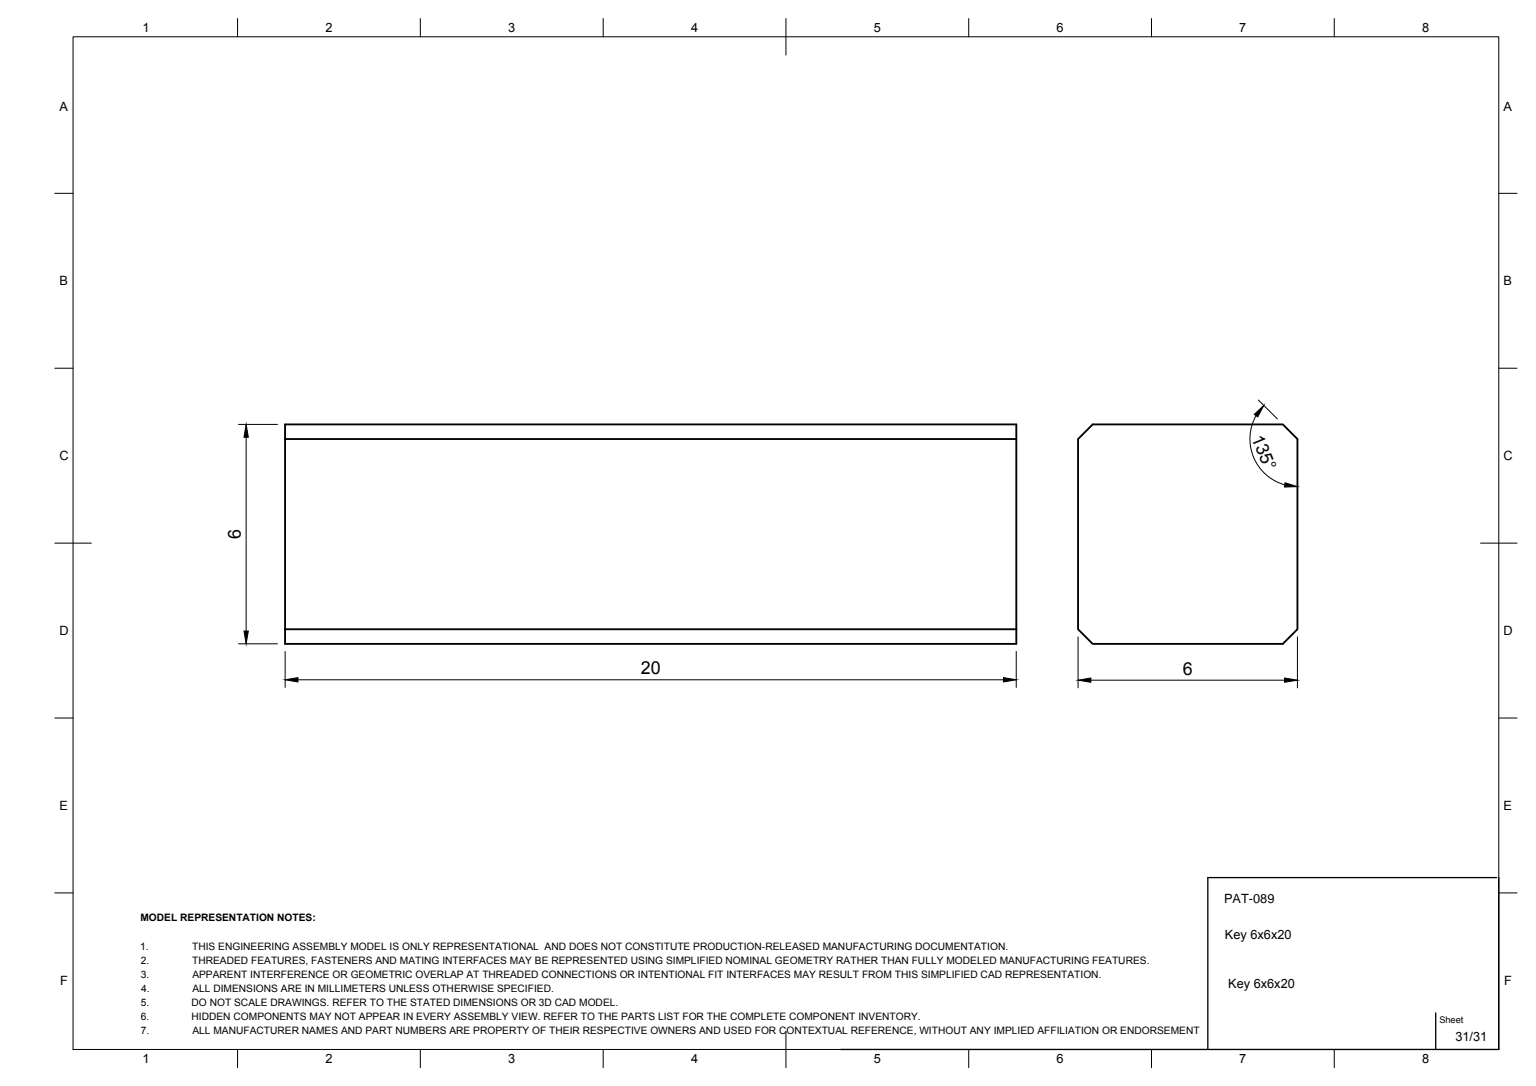
ISO-10303-21;
HEADER;
/* Generated by software containing ST-Developer
 * from STEP Tools, Inc. (www.steptools.com) 
 */

FILE_DESCRIPTION(
/* description */ ('Rotary union on bearing shaft'),
/* implementation_level */ '2;1');

FILE_NAME(
/* name */ 'Key 6x6x20.step',
/* time_stamp */ '2026-10-28T03:24:01-07:00',
/* author */ (''),
/* organization */ (''),
/* preprocessor_version */ 'ST-DEVELOPER v20.2',
/* originating_system */ 'Autodesk Translation Framework v15.17.0.0',
/* authorisation */ '');

FILE_SCHEMA (('AUTOMOTIVE_DESIGN { 1 0 10303 214 3 1 1 }'));
ENDSEC;

DATA;
#10=MECHANICAL_DESIGN_GEOMETRIC_PRESENTATION_REPRESENTATION('',(#346),#9448);
#284=SHAPE_REPRESENTATION_RELATIONSHIP('SRR','None',#9586,#311);
#311=ADVANCED_BREP_SHAPE_REPRESENTATION('',(#379),#9446);
#346=STYLED_ITEM('',(#9778),#379);
#379=MANIFOLD_SOLID_BREP('Body1',#4903);
#635=PLANE('',#5781);
#636=PLANE('',#5782);
#637=PLANE('',#5783);
#638=PLANE('',#5784);
#639=PLANE('',#5785);
#640=PLANE('',#5786);
#641=PLANE('',#5787);
#642=PLANE('',#5788);
#643=PLANE('',#5789);
#644=PLANE('',#5790);
#928=FACE_OUTER_BOUND('',#1333,.T.);
#929=FACE_OUTER_BOUND('',#1334,.T.);
#930=FACE_OUTER_BOUND('',#1335,.T.);
#931=FACE_OUTER_BOUND('',#1336,.T.);
#932=FACE_OUTER_BOUND('',#1337,.T.);
#933=FACE_OUTER_BOUND('',#1338,.T.);
#934=FACE_OUTER_BOUND('',#1339,.T.);
#935=FACE_OUTER_BOUND('',#1340,.T.);
#936=FACE_OUTER_BOUND('',#1341,.T.);
#937=FACE_OUTER_BOUND('',#1342,.T.);
#1333=EDGE_LOOP('',(#4367,#4368,#4369,#4370,#4371,#4372,#4373,#4374));
#1334=EDGE_LOOP('',(#4375,#4376,#4377,#4378));
#1335=EDGE_LOOP('',(#4379,#4380,#4381,#4382));
#1336=EDGE_LOOP('',(#4383,#4384,#4385,#4386));
#1337=EDGE_LOOP('',(#4387,#4388,#4389,#4390));
#1338=EDGE_LOOP('',(#4391,#4392,#4393,#4394,#4395,#4396,#4397,#4398));
#1339=EDGE_LOOP('',(#4399,#4400,#4401,#4402));
#1340=EDGE_LOOP('',(#4403,#4404,#4405,#4406));
#1341=EDGE_LOOP('',(#4407,#4408,#4409,#4410));
#1342=EDGE_LOOP('',(#4411,#4412,#4413,#4414));
#1633=LINE('',#9257,#1953);
#1634=LINE('',#9259,#1954);
#1635=LINE('',#9261,#1955);
#1636=LINE('',#9263,#1956);
#1637=LINE('',#9265,#1957);
#1638=LINE('',#9267,#1958);
#1639=LINE('',#9269,#1959);
#1640=LINE('',#9270,#1960);
#1641=LINE('',#9273,#1961);
#1642=LINE('',#9275,#1962);
#1643=LINE('',#9276,#1963);
#1644=LINE('',#9279,#1964);
#1645=LINE('',#9280,#1965);
#1646=LINE('',#9283,#1966);
#1647=LINE('',#9284,#1967);
#1648=LINE('',#9287,#1968);
#1649=LINE('',#9288,#1969);
#1650=LINE('',#9292,#1970);
#1651=LINE('',#9293,#1971);
#1652=LINE('',#9295,#1972);
#1653=LINE('',#9296,#1973);
#1654=LINE('',#9298,#1974);
#1655=LINE('',#9300,#1975);
#1656=LINE('',#9302,#1976);
#1953=VECTOR('',#7256,1.);
#1954=VECTOR('',#7257,1.);
#1955=VECTOR('',#7258,1.);
#1956=VECTOR('',#7259,1.);
#1957=VECTOR('',#7260,1.);
#1958=VECTOR('',#7261,1.);
#1959=VECTOR('',#7262,1.);
#1960=VECTOR('',#7263,1.);
#1961=VECTOR('',#7266,1.);
#1962=VECTOR('',#7267,1.);
#1963=VECTOR('',#7268,1.);
#1964=VECTOR('',#7271,1.);
#1965=VECTOR('',#7272,1.);
#1966=VECTOR('',#7275,1.);
#1967=VECTOR('',#7276,1.);
#1968=VECTOR('',#7279,1.);
#1969=VECTOR('',#7280,1.);
#1970=VECTOR('',#7283,1.);
#1971=VECTOR('',#7284,1.);
#1972=VECTOR('',#7285,1.);
#1973=VECTOR('',#7286,1.);
#1974=VECTOR('',#7289,1.);
#1975=VECTOR('',#7292,1.);
#1976=VECTOR('',#7295,1.);
#2625=VERTEX_POINT('',#9255);
#2626=VERTEX_POINT('',#9256);
#2627=VERTEX_POINT('',#9258);
#2628=VERTEX_POINT('',#9260);
#2629=VERTEX_POINT('',#9262);
#2630=VERTEX_POINT('',#9264);
#2631=VERTEX_POINT('',#9266);
#2632=VERTEX_POINT('',#9268);
#2633=VERTEX_POINT('',#9272);
#2634=VERTEX_POINT('',#9274);
#2635=VERTEX_POINT('',#9278);
#2636=VERTEX_POINT('',#9282);
#2637=VERTEX_POINT('',#9286);
#2638=VERTEX_POINT('',#9290);
#2639=VERTEX_POINT('',#9291);
#2640=VERTEX_POINT('',#9294);
#3211=EDGE_CURVE('',#2625,#2626,#1633,.T.);
#3212=EDGE_CURVE('',#2627,#2625,#1634,.T.);
#3213=EDGE_CURVE('',#2628,#2627,#1635,.T.);
#3214=EDGE_CURVE('',#2629,#2628,#1636,.T.);
#3215=EDGE_CURVE('',#2630,#2629,#1637,.T.);
#3216=EDGE_CURVE('',#2631,#2630,#1638,.T.);
#3217=EDGE_CURVE('',#2632,#2631,#1639,.T.);
#3218=EDGE_CURVE('',#2626,#2632,#1640,.T.);
#3219=EDGE_CURVE('',#2629,#2633,#1641,.T.);
#3220=EDGE_CURVE('',#2633,#2634,#1642,.T.);
#3221=EDGE_CURVE('',#2634,#2630,#1643,.T.);
#3222=EDGE_CURVE('',#2635,#2628,#1644,.T.);
#3223=EDGE_CURVE('',#2635,#2633,#1645,.T.);
#3224=EDGE_CURVE('',#2627,#2636,#1646,.T.);
#3225=EDGE_CURVE('',#2636,#2635,#1647,.T.);
#3226=EDGE_CURVE('',#2637,#2625,#1648,.T.);
#3227=EDGE_CURVE('',#2637,#2636,#1649,.T.);
#3228=EDGE_CURVE('',#2638,#2639,#1650,.T.);
#3229=EDGE_CURVE('',#2634,#2638,#1651,.T.);
#3230=EDGE_CURVE('',#2640,#2637,#1652,.T.);
#3231=EDGE_CURVE('',#2639,#2640,#1653,.T.);
#3232=EDGE_CURVE('',#2631,#2638,#1654,.T.);
#3233=EDGE_CURVE('',#2626,#2640,#1655,.T.);
#3234=EDGE_CURVE('',#2639,#2632,#1656,.T.);
#4367=ORIENTED_EDGE('',*,*,#3211,.F.);
#4368=ORIENTED_EDGE('',*,*,#3212,.F.);
#4369=ORIENTED_EDGE('',*,*,#3213,.F.);
#4370=ORIENTED_EDGE('',*,*,#3214,.F.);
#4371=ORIENTED_EDGE('',*,*,#3215,.F.);
#4372=ORIENTED_EDGE('',*,*,#3216,.F.);
#4373=ORIENTED_EDGE('',*,*,#3217,.F.);
#4374=ORIENTED_EDGE('',*,*,#3218,.F.);
#4375=ORIENTED_EDGE('',*,*,#3215,.T.);
#4376=ORIENTED_EDGE('',*,*,#3219,.T.);
#4377=ORIENTED_EDGE('',*,*,#3220,.T.);
#4378=ORIENTED_EDGE('',*,*,#3221,.T.);
#4379=ORIENTED_EDGE('',*,*,#3214,.T.);
#4380=ORIENTED_EDGE('',*,*,#3222,.F.);
#4381=ORIENTED_EDGE('',*,*,#3223,.T.);
#4382=ORIENTED_EDGE('',*,*,#3219,.F.);
#4383=ORIENTED_EDGE('',*,*,#3213,.T.);
#4384=ORIENTED_EDGE('',*,*,#3224,.T.);
#4385=ORIENTED_EDGE('',*,*,#3225,.T.);
#4386=ORIENTED_EDGE('',*,*,#3222,.T.);
#4387=ORIENTED_EDGE('',*,*,#3212,.T.);
#4388=ORIENTED_EDGE('',*,*,#3226,.F.);
#4389=ORIENTED_EDGE('',*,*,#3227,.T.);
#4390=ORIENTED_EDGE('',*,*,#3224,.F.);
#4391=ORIENTED_EDGE('',*,*,#3228,.F.);
#4392=ORIENTED_EDGE('',*,*,#3229,.F.);
#4393=ORIENTED_EDGE('',*,*,#3220,.F.);
#4394=ORIENTED_EDGE('',*,*,#3223,.F.);
#4395=ORIENTED_EDGE('',*,*,#3225,.F.);
#4396=ORIENTED_EDGE('',*,*,#3227,.F.);
#4397=ORIENTED_EDGE('',*,*,#3230,.F.);
#4398=ORIENTED_EDGE('',*,*,#3231,.F.);
#4399=ORIENTED_EDGE('',*,*,#3216,.T.);
#4400=ORIENTED_EDGE('',*,*,#3221,.F.);
#4401=ORIENTED_EDGE('',*,*,#3229,.T.);
#4402=ORIENTED_EDGE('',*,*,#3232,.F.);
#4403=ORIENTED_EDGE('',*,*,#3211,.T.);
#4404=ORIENTED_EDGE('',*,*,#3233,.T.);
#4405=ORIENTED_EDGE('',*,*,#3230,.T.);
#4406=ORIENTED_EDGE('',*,*,#3226,.T.);
#4407=ORIENTED_EDGE('',*,*,#3217,.T.);
#4408=ORIENTED_EDGE('',*,*,#3232,.T.);
#4409=ORIENTED_EDGE('',*,*,#3228,.T.);
#4410=ORIENTED_EDGE('',*,*,#3234,.T.);
#4411=ORIENTED_EDGE('',*,*,#3218,.T.);
#4412=ORIENTED_EDGE('',*,*,#3234,.F.);
#4413=ORIENTED_EDGE('',*,*,#3231,.T.);
#4414=ORIENTED_EDGE('',*,*,#3233,.F.);
#4841=ADVANCED_FACE('',(#928),#635,.F.);
#4842=ADVANCED_FACE('',(#929),#636,.T.);
#4843=ADVANCED_FACE('',(#930),#637,.T.);
#4844=ADVANCED_FACE('',(#931),#638,.T.);
#4845=ADVANCED_FACE('',(#932),#639,.T.);
#4846=ADVANCED_FACE('',(#933),#640,.T.);
#4847=ADVANCED_FACE('',(#934),#641,.F.);
#4848=ADVANCED_FACE('',(#935),#642,.T.);
#4849=ADVANCED_FACE('',(#936),#643,.T.);
#4850=ADVANCED_FACE('',(#937),#644,.T.);
#4903=CLOSED_SHELL('',(#4841,#4842,#4843,#4844,#4845,#4846,#4847,#4848,
#4849,#4850));
#5780=AXIS2_PLACEMENT_3D('',#9253,#7252,#7253);
#5781=AXIS2_PLACEMENT_3D('',#9254,#7254,#7255);
#5782=AXIS2_PLACEMENT_3D('',#9271,#7264,#7265);
#5783=AXIS2_PLACEMENT_3D('',#9277,#7269,#7270);
#5784=AXIS2_PLACEMENT_3D('',#9281,#7273,#7274);
#5785=AXIS2_PLACEMENT_3D('',#9285,#7277,#7278);
#5786=AXIS2_PLACEMENT_3D('',#9289,#7281,#7282);
#5787=AXIS2_PLACEMENT_3D('',#9297,#7287,#7288);
#5788=AXIS2_PLACEMENT_3D('',#9299,#7290,#7291);
#5789=AXIS2_PLACEMENT_3D('',#9301,#7293,#7294);
#5790=AXIS2_PLACEMENT_3D('',#9303,#7296,#7297);
#7252=DIRECTION('axis',(0.,0.,1.));
#7253=DIRECTION('refdir',(1.,0.,0.));
#7254=DIRECTION('center_axis',(1.,0.,0.));
#7255=DIRECTION('ref_axis',(0.,0.,-1.));
#7256=DIRECTION('',(0.,-0.707106781186547,-0.707106781186548));
#7257=DIRECTION('',(0.,-1.,0.));
#7258=DIRECTION('',(0.,-0.707106781186547,0.707106781186548));
#7259=DIRECTION('',(0.,0.,1.));
#7260=DIRECTION('',(0.,0.707106781186547,0.707106781186548));
#7261=DIRECTION('',(0.,1.,0.));
#7262=DIRECTION('',(0.,0.707106781186547,-0.707106781186548));
#7263=DIRECTION('',(0.,0.,-1.));
#7264=DIRECTION('center_axis',(0.,0.707106781186548,-0.707106781186547));
#7265=DIRECTION('ref_axis',(-1.,0.,0.));
#7266=DIRECTION('',(1.,0.,0.));
#7267=DIRECTION('',(0.,-0.707106781186547,-0.707106781186548));
#7268=DIRECTION('',(-1.,0.,0.));
#7269=DIRECTION('center_axis',(0.,1.,0.));
#7270=DIRECTION('ref_axis',(-1.,0.,0.));
#7271=DIRECTION('',(-1.,0.,0.));
#7272=DIRECTION('',(0.,0.,-1.));
#7273=DIRECTION('center_axis',(0.,0.707106781186548,0.707106781186547));
#7274=DIRECTION('ref_axis',(1.,0.,0.));
#7275=DIRECTION('',(1.,0.,0.));
#7276=DIRECTION('',(0.,0.707106781186547,-0.707106781186548));
#7277=DIRECTION('center_axis',(0.,0.,1.));
#7278=DIRECTION('ref_axis',(1.,0.,0.));
#7279=DIRECTION('',(-1.,0.,0.));
#7280=DIRECTION('',(0.,1.,0.));
#7281=DIRECTION('center_axis',(1.,0.,0.));
#7282=DIRECTION('ref_axis',(0.,0.,-1.));
#7283=DIRECTION('',(0.,-0.707106781186547,0.707106781186548));
#7284=DIRECTION('',(0.,-1.,0.));
#7285=DIRECTION('',(0.,0.707106781186547,0.707106781186548));
#7286=DIRECTION('',(0.,0.,1.));
#7287=DIRECTION('center_axis',(0.,0.,1.));
#7288=DIRECTION('ref_axis',(1.,0.,0.));
#7289=DIRECTION('',(1.,0.,0.));
#7290=DIRECTION('center_axis',(0.,-0.707106781186548,0.707106781186547));
#7291=DIRECTION('ref_axis',(1.,0.,0.));
#7292=DIRECTION('',(1.,0.,0.));
#7293=DIRECTION('center_axis',(0.,-0.707106781186548,-0.707106781186547));
#7294=DIRECTION('ref_axis',(-1.,0.,0.));
#7295=DIRECTION('',(-1.,0.,0.));
#7296=DIRECTION('center_axis',(0.,-1.,0.));
#7297=DIRECTION('ref_axis',(1.,0.,0.));
#9253=CARTESIAN_POINT('',(0.,0.,0.));
#9254=CARTESIAN_POINT('Origin',(-1.,0.,0.35));
#9255=CARTESIAN_POINT('',(-1.,-0.26,0.6));
#9256=CARTESIAN_POINT('',(-1.,-0.3,0.56));
#9257=CARTESIAN_POINT('',(-1.,-0.2675,0.5925));
#9258=CARTESIAN_POINT('',(-1.,0.26,0.6));
#9259=CARTESIAN_POINT('',(-1.,0.,0.6));
#9260=CARTESIAN_POINT('',(-1.,0.3,0.56));
#9261=CARTESIAN_POINT('',(-1.,0.2675,0.5925));
#9262=CARTESIAN_POINT('',(-1.,0.3,0.04));
#9263=CARTESIAN_POINT('',(-1.,0.3,0.175));
#9264=CARTESIAN_POINT('',(-1.,0.26,0.));
#9265=CARTESIAN_POINT('',(-1.,0.2925,0.0325));
#9266=CARTESIAN_POINT('',(-1.,-0.26,0.));
#9267=CARTESIAN_POINT('',(-1.,0.,0.));
#9268=CARTESIAN_POINT('',(-1.,-0.3,0.04));
#9269=CARTESIAN_POINT('',(-1.,-0.2925,0.0325));
#9270=CARTESIAN_POINT('',(-1.,-0.3,0.175));
#9271=CARTESIAN_POINT('Origin',(0.75,0.28,0.02));
#9272=CARTESIAN_POINT('',(1.,0.3,0.04));
#9273=CARTESIAN_POINT('',(0.75,0.3,0.04));
#9274=CARTESIAN_POINT('',(1.,0.26,0.));
#9275=CARTESIAN_POINT('',(1.,0.2925,0.0325));
#9276=CARTESIAN_POINT('',(0.75,0.26,0.));
#9277=CARTESIAN_POINT('Origin',(1.5,0.3,0.));
#9278=CARTESIAN_POINT('',(1.,0.3,0.56));
#9279=CARTESIAN_POINT('',(0.75,0.3,0.56));
#9280=CARTESIAN_POINT('',(1.,0.3,0.175));
#9281=CARTESIAN_POINT('Origin',(0.75,0.28,0.58));
#9282=CARTESIAN_POINT('',(1.,0.26,0.6));
#9283=CARTESIAN_POINT('',(0.75,0.26,0.6));
#9284=CARTESIAN_POINT('',(1.,0.2675,0.5925));
#9285=CARTESIAN_POINT('Origin',(0.,0.,0.6));
#9286=CARTESIAN_POINT('',(1.,-0.26,0.6));
#9287=CARTESIAN_POINT('',(-0.75,-0.26,0.6));
#9288=CARTESIAN_POINT('',(1.,0.,0.6));
#9289=CARTESIAN_POINT('Origin',(1.,0.,0.35));
#9290=CARTESIAN_POINT('',(1.,-0.26,0.));
#9291=CARTESIAN_POINT('',(1.,-0.3,0.04));
#9292=CARTESIAN_POINT('',(1.,-0.2925,0.0325));
#9293=CARTESIAN_POINT('',(1.,0.,0.));
#9294=CARTESIAN_POINT('',(1.,-0.3,0.56));
#9295=CARTESIAN_POINT('',(1.,-0.2675,0.5925));
#9296=CARTESIAN_POINT('',(1.,-0.3,0.175));
#9297=CARTESIAN_POINT('Origin',(0.,0.,0.));
#9298=CARTESIAN_POINT('',(-0.75,-0.26,0.));
#9299=CARTESIAN_POINT('Origin',(-0.75,-0.28,0.58));
#9300=CARTESIAN_POINT('',(-0.75,-0.3,0.56));
#9301=CARTESIAN_POINT('Origin',(-0.75,-0.28,0.02));
#9302=CARTESIAN_POINT('',(-0.75,-0.3,0.04));
#9303=CARTESIAN_POINT('Origin',(-1.5,-0.3,0.));
#9414=UNCERTAINTY_MEASURE_WITH_UNIT(LENGTH_MEASURE(0.001),#9449,
'DISTANCE_ACCURACY_VALUE',
'Maximum model space distance between geometric entities at asserted c
onnectivities');
#9416=UNCERTAINTY_MEASURE_WITH_UNIT(LENGTH_MEASURE(0.001),#9449,
'DISTANCE_ACCURACY_VALUE',
'Maximum model space distance between geometric entities at asserted c
onnectivities');
#9446=(
GEOMETRIC_REPRESENTATION_CONTEXT(3)
GLOBAL_UNCERTAINTY_ASSIGNED_CONTEXT((#9414))
GLOBAL_UNIT_ASSIGNED_CONTEXT((#9449,#9451,#9452))
REPRESENTATION_CONTEXT('','3D')
);
#9448=(
GEOMETRIC_REPRESENTATION_CONTEXT(3)
GLOBAL_UNCERTAINTY_ASSIGNED_CONTEXT((#9416))
GLOBAL_UNIT_ASSIGNED_CONTEXT((#9449,#9451,#9452))
REPRESENTATION_CONTEXT('','3D')
);
#9449=(
LENGTH_UNIT()
NAMED_UNIT(*)
SI_UNIT(.CENTI.,.METRE.)
);
#9451=(
NAMED_UNIT(*)
PLANE_ANGLE_UNIT()
SI_UNIT($,.RADIAN.)
);
#9452=(
NAMED_UNIT(*)
SI_UNIT($,.STERADIAN.)
SOLID_ANGLE_UNIT()
);
#9482=SHAPE_DEFINITION_REPRESENTATION(#9544,#9586);
#9544=PRODUCT_DEFINITION_SHAPE('',$,#9618);
#9586=SHAPE_REPRESENTATION('',(#5780),#9446);
#9588=PRODUCT_DEFINITION_CONTEXT('part definition',#9683,'design');
#9618=PRODUCT_DEFINITION('Key 6x6x20','Key 6x6x20',#9649,#9588);
#9649=PRODUCT_DEFINITION_FORMATION('',$,#9714);
#9683=APPLICATION_CONTEXT(
'Core Data for Automotive Mechanical Design Process');
#9684=PRODUCT_CONTEXT('part definition',#9683,'mechanical');
#9714=PRODUCT('Key 6x6x20','Key 6x6x20','Key 6x6x20',(#9684));
#9772=COLOUR_RGB('Grey',0.48,0.52,0.57);
#9773=FILL_AREA_STYLE_COLOUR('',#9772);
#9774=FILL_AREA_STYLE('',(#9773));
#9775=SURFACE_STYLE_FILL_AREA(#9774);
#9776=SURFACE_SIDE_STYLE('',(#9775));
#9777=SURFACE_STYLE_USAGE(.BOTH.,#9776);
#9778=PRESENTATION_STYLE_ASSIGNMENT((#9777));
ENDSEC;
END-ISO-10303-21;
